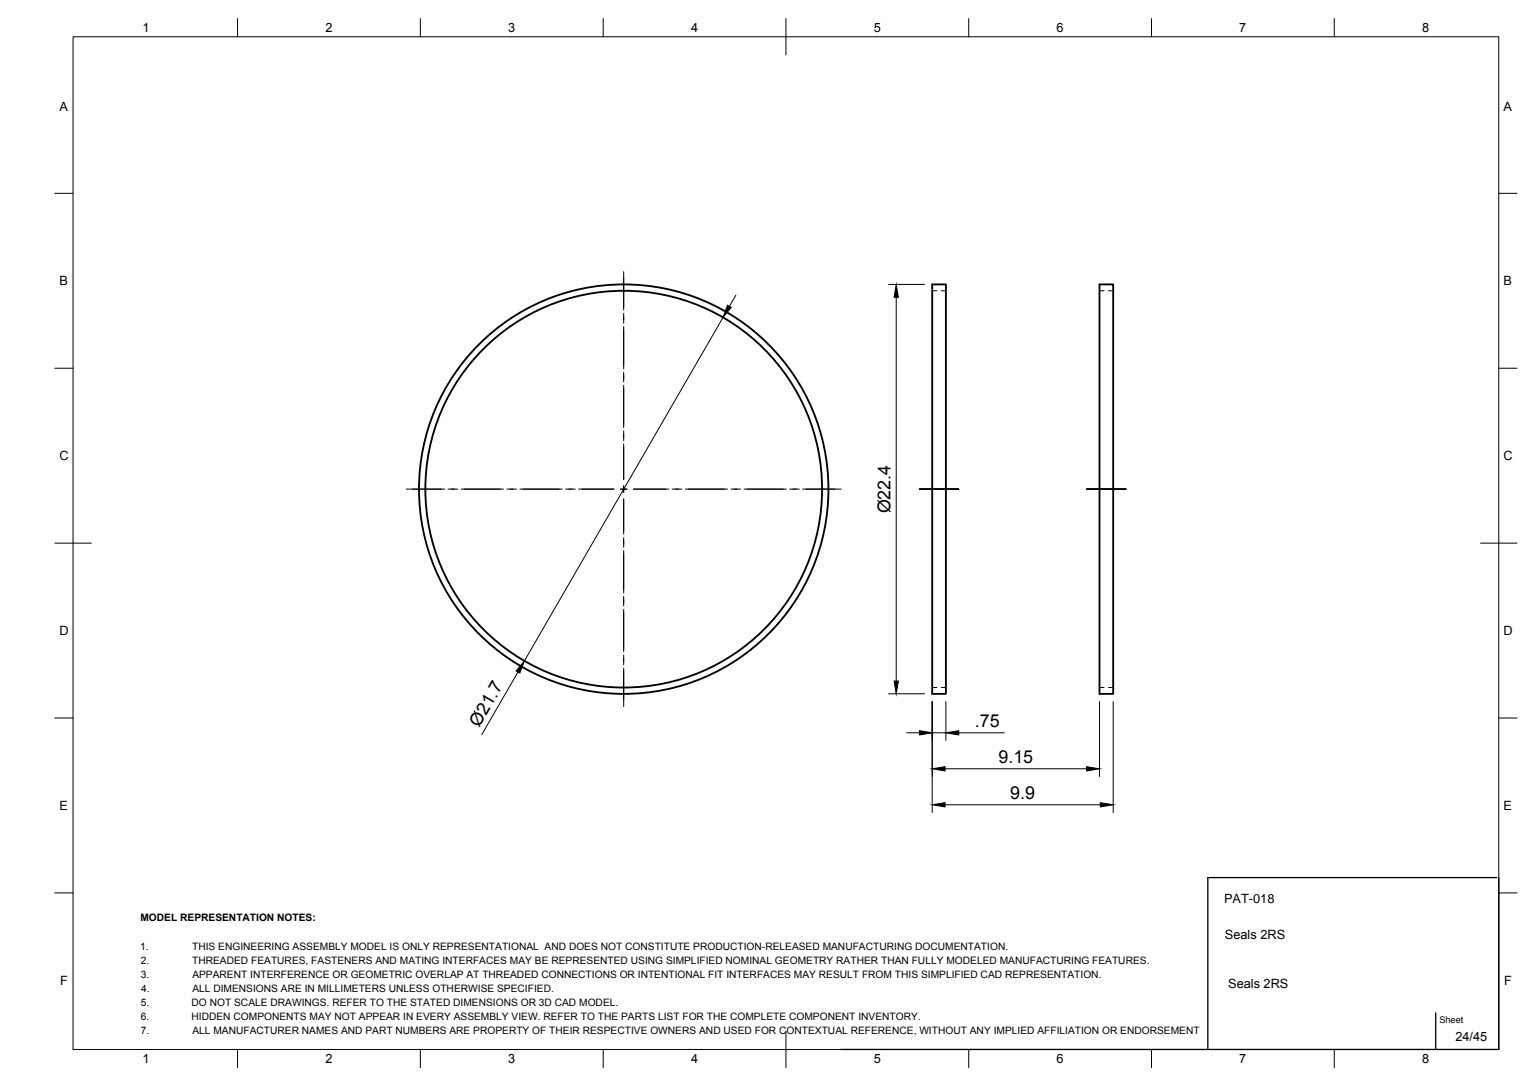
ISO-10303-21;
HEADER;
/* Generated by software containing ST-Developer
 * from STEP Tools, Inc. (www.steptools.com) 
 */

FILE_DESCRIPTION(
/* description */ ('Cam-driven reciprocating slide'),
/* implementation_level */ '2;1');

FILE_NAME(
/* name */ 'Seals 2RS.step',
/* time_stamp */ '2026-10-28T03:25:20-07:00',
/* author */ (''),
/* organization */ (''),
/* preprocessor_version */ 'ST-DEVELOPER v20.2',
/* originating_system */ 'Autodesk Translation Framework v15.17.0.0',
/* authorisation */ '');

FILE_SCHEMA (('AUTOMOTIVE_DESIGN { 1 0 10303 214 3 1 1 }'));
ENDSEC;

DATA;
#10=MECHANICAL_DESIGN_GEOMETRIC_PRESENTATION_REPRESENTATION('',(#445,#446),#13277);
#365=SHAPE_REPRESENTATION_RELATIONSHIP('SRR','None',#13459,#402);
#402=ADVANCED_BREP_SHAPE_REPRESENTATION('',(#489,#490),#13254);
#445=STYLED_ITEM('',(#13720),#489);
#446=STYLED_ITEM('',(#13720),#490);
#489=MANIFOLD_SOLID_BREP('Body1',#6421);
#490=MANIFOLD_SOLID_BREP('Body2',#6422);
#623=FACE_BOUND('',#1588,.T.);
#624=FACE_BOUND('',#1591,.T.);
#625=FACE_BOUND('',#1594,.T.);
#626=FACE_BOUND('',#1597,.T.);
#776=PLANE('',#7261);
#777=PLANE('',#7266);
#778=PLANE('',#7269);
#779=PLANE('',#7274);
#1092=FACE_OUTER_BOUND('',#1587,.T.);
#1093=FACE_OUTER_BOUND('',#1589,.T.);
#1094=FACE_OUTER_BOUND('',#1590,.T.);
#1095=FACE_OUTER_BOUND('',#1592,.T.);
#1096=FACE_OUTER_BOUND('',#1593,.T.);
#1097=FACE_OUTER_BOUND('',#1595,.T.);
#1098=FACE_OUTER_BOUND('',#1596,.T.);
#1099=FACE_OUTER_BOUND('',#1598,.T.);
#1587=EDGE_LOOP('',(#5182));
#1588=EDGE_LOOP('',(#5183));
#1589=EDGE_LOOP('',(#5184,#5185,#5186,#5187));
#1590=EDGE_LOOP('',(#5188));
#1591=EDGE_LOOP('',(#5189));
#1592=EDGE_LOOP('',(#5190,#5191,#5192,#5193));
#1593=EDGE_LOOP('',(#5194));
#1594=EDGE_LOOP('',(#5195));
#1595=EDGE_LOOP('',(#5196,#5197,#5198,#5199));
#1596=EDGE_LOOP('',(#5200));
#1597=EDGE_LOOP('',(#5201));
#1598=EDGE_LOOP('',(#5202,#5203,#5204,#5205));
#2044=LINE('',#12329,#2483);
#2045=LINE('',#12334,#2484);
#2046=LINE('',#12343,#2485);
#2047=LINE('',#12348,#2486);
#2483=VECTOR('',#8706,1.119765);
#2484=VECTOR('',#8713,1.085235);
#2485=VECTOR('',#8724,1.119765);
#2486=VECTOR('',#8731,1.085235);
#2908=CIRCLE('',#7262,1.119765);
#2909=CIRCLE('',#7263,1.085235);
#2910=CIRCLE('',#7265,1.119765);
#2911=CIRCLE('',#7267,1.085235);
#2912=CIRCLE('',#7270,1.119765);
#2913=CIRCLE('',#7271,1.085235);
#2914=CIRCLE('',#7273,1.119765);
#2915=CIRCLE('',#7275,1.085235);
#3325=VERTEX_POINT('',#12322);
#3326=VERTEX_POINT('',#12324);
#3327=VERTEX_POINT('',#12327);
#3328=VERTEX_POINT('',#12331);
#3329=VERTEX_POINT('',#12336);
#3330=VERTEX_POINT('',#12338);
#3331=VERTEX_POINT('',#12341);
#3332=VERTEX_POINT('',#12345);
#3981=EDGE_CURVE('',#3325,#3325,#2908,.T.);
#3982=EDGE_CURVE('',#3326,#3326,#2909,.T.);
#3983=EDGE_CURVE('',#3327,#3327,#2910,.T.);
#3984=EDGE_CURVE('',#3327,#3325,#2044,.T.);
#3985=EDGE_CURVE('',#3328,#3328,#2911,.T.);
#3986=EDGE_CURVE('',#3328,#3326,#2045,.T.);
#3987=EDGE_CURVE('',#3329,#3329,#2912,.T.);
#3988=EDGE_CURVE('',#3330,#3330,#2913,.T.);
#3989=EDGE_CURVE('',#3331,#3331,#2914,.T.);
#3990=EDGE_CURVE('',#3331,#3329,#2046,.T.);
#3991=EDGE_CURVE('',#3332,#3332,#2915,.T.);
#3992=EDGE_CURVE('',#3332,#3330,#2047,.T.);
#5182=ORIENTED_EDGE('',*,*,#3981,.F.);
#5183=ORIENTED_EDGE('',*,*,#3982,.T.);
#5184=ORIENTED_EDGE('',*,*,#3983,.F.);
#5185=ORIENTED_EDGE('',*,*,#3984,.T.);
#5186=ORIENTED_EDGE('',*,*,#3981,.T.);
#5187=ORIENTED_EDGE('',*,*,#3984,.F.);
#5188=ORIENTED_EDGE('',*,*,#3983,.T.);
#5189=ORIENTED_EDGE('',*,*,#3985,.F.);
#5190=ORIENTED_EDGE('',*,*,#3985,.T.);
#5191=ORIENTED_EDGE('',*,*,#3986,.T.);
#5192=ORIENTED_EDGE('',*,*,#3982,.F.);
#5193=ORIENTED_EDGE('',*,*,#3986,.F.);
#5194=ORIENTED_EDGE('',*,*,#3987,.F.);
#5195=ORIENTED_EDGE('',*,*,#3988,.T.);
#5196=ORIENTED_EDGE('',*,*,#3989,.F.);
#5197=ORIENTED_EDGE('',*,*,#3990,.T.);
#5198=ORIENTED_EDGE('',*,*,#3987,.T.);
#5199=ORIENTED_EDGE('',*,*,#3990,.F.);
#5200=ORIENTED_EDGE('',*,*,#3989,.T.);
#5201=ORIENTED_EDGE('',*,*,#3991,.F.);
#5202=ORIENTED_EDGE('',*,*,#3991,.T.);
#5203=ORIENTED_EDGE('',*,*,#3992,.T.);
#5204=ORIENTED_EDGE('',*,*,#3988,.F.);
#5205=ORIENTED_EDGE('',*,*,#3992,.F.);
#5967=CYLINDRICAL_SURFACE('',#7264,1.119765);
#5968=CYLINDRICAL_SURFACE('',#7268,1.085235);
#5969=CYLINDRICAL_SURFACE('',#7272,1.119765);
#5970=CYLINDRICAL_SURFACE('',#7276,1.085235);
#6210=ADVANCED_FACE('',(#1092,#623),#776,.T.);
#6211=ADVANCED_FACE('',(#1093),#5967,.T.);
#6212=ADVANCED_FACE('',(#1094,#624),#777,.T.);
#6213=ADVANCED_FACE('',(#1095),#5968,.F.);
#6214=ADVANCED_FACE('',(#1096,#625),#778,.T.);
#6215=ADVANCED_FACE('',(#1097),#5969,.T.);
#6216=ADVANCED_FACE('',(#1098,#626),#779,.T.);
#6217=ADVANCED_FACE('',(#1099),#5970,.F.);
#6421=CLOSED_SHELL('',(#6210,#6211,#6212,#6213));
#6422=CLOSED_SHELL('',(#6214,#6215,#6216,#6217));
#7260=AXIS2_PLACEMENT_3D('',#12320,#8694,#8695);
#7261=AXIS2_PLACEMENT_3D('',#12321,#8696,#8697);
#7262=AXIS2_PLACEMENT_3D('',#12323,#8698,#8699);
#7263=AXIS2_PLACEMENT_3D('',#12325,#8700,#8701);
#7264=AXIS2_PLACEMENT_3D('',#12326,#8702,#8703);
#7265=AXIS2_PLACEMENT_3D('',#12328,#8704,#8705);
#7266=AXIS2_PLACEMENT_3D('',#12330,#8707,#8708);
#7267=AXIS2_PLACEMENT_3D('',#12332,#8709,#8710);
#7268=AXIS2_PLACEMENT_3D('',#12333,#8711,#8712);
#7269=AXIS2_PLACEMENT_3D('',#12335,#8714,#8715);
#7270=AXIS2_PLACEMENT_3D('',#12337,#8716,#8717);
#7271=AXIS2_PLACEMENT_3D('',#12339,#8718,#8719);
#7272=AXIS2_PLACEMENT_3D('',#12340,#8720,#8721);
#7273=AXIS2_PLACEMENT_3D('',#12342,#8722,#8723);
#7274=AXIS2_PLACEMENT_3D('',#12344,#8725,#8726);
#7275=AXIS2_PLACEMENT_3D('',#12346,#8727,#8728);
#7276=AXIS2_PLACEMENT_3D('',#12347,#8729,#8730);
#8694=DIRECTION('axis',(0.,0.,1.));
#8695=DIRECTION('refdir',(1.,0.,0.));
#8696=DIRECTION('center_axis',(0.,1.,0.));
#8697=DIRECTION('ref_axis',(0.,0.,1.));
#8698=DIRECTION('center_axis',(0.,-1.,0.));
#8699=DIRECTION('ref_axis',(1.,0.,0.));
#8700=DIRECTION('center_axis',(0.,-1.,0.));
#8701=DIRECTION('ref_axis',(1.,0.,0.));
#8702=DIRECTION('center_axis',(0.,-1.,0.));
#8703=DIRECTION('ref_axis',(1.,0.,0.));
#8704=DIRECTION('center_axis',(0.,-1.,0.));
#8705=DIRECTION('ref_axis',(1.,0.,0.));
#8706=DIRECTION('',(0.,1.,0.));
#8707=DIRECTION('center_axis',(0.,-1.,0.));
#8708=DIRECTION('ref_axis',(0.,0.,-1.));
#8709=DIRECTION('center_axis',(0.,-1.,0.));
#8710=DIRECTION('ref_axis',(1.,0.,0.));
#8711=DIRECTION('center_axis',(0.,-1.,0.));
#8712=DIRECTION('ref_axis',(1.,0.,0.));
#8713=DIRECTION('',(0.,1.,0.));
#8714=DIRECTION('center_axis',(0.,1.,0.));
#8715=DIRECTION('ref_axis',(0.,0.,1.));
#8716=DIRECTION('center_axis',(0.,-1.,0.));
#8717=DIRECTION('ref_axis',(1.,0.,0.));
#8718=DIRECTION('center_axis',(0.,-1.,0.));
#8719=DIRECTION('ref_axis',(1.,0.,0.));
#8720=DIRECTION('center_axis',(0.,-1.,0.));
#8721=DIRECTION('ref_axis',(1.,0.,0.));
#8722=DIRECTION('center_axis',(0.,-1.,0.));
#8723=DIRECTION('ref_axis',(1.,0.,0.));
#8724=DIRECTION('',(0.,1.,0.));
#8725=DIRECTION('center_axis',(0.,-1.,0.));
#8726=DIRECTION('ref_axis',(0.,0.,-1.));
#8727=DIRECTION('center_axis',(0.,-1.,0.));
#8728=DIRECTION('ref_axis',(1.,0.,0.));
#8729=DIRECTION('center_axis',(0.,-1.,0.));
#8730=DIRECTION('ref_axis',(1.,0.,0.));
#8731=DIRECTION('',(0.,1.,0.));
#12320=CARTESIAN_POINT('',(0.,0.,0.));
#12321=CARTESIAN_POINT('Origin',(1.119765,0.495,0.));
#12322=CARTESIAN_POINT('',(-1.119765,0.495,-1.37131662304724E-16));
#12323=CARTESIAN_POINT('Origin',(0.,0.495,0.));
#12324=CARTESIAN_POINT('',(-1.085235,0.495,-1.32902956907268E-16));
#12325=CARTESIAN_POINT('Origin',(0.,0.495,0.));
#12326=CARTESIAN_POINT('Origin',(0.,0.4575,0.));
#12327=CARTESIAN_POINT('',(-1.119765,0.42,-1.37131662304724E-16));
#12328=CARTESIAN_POINT('Origin',(0.,0.42,0.));
#12329=CARTESIAN_POINT('',(-1.119765,0.4575,-1.37131662304724E-16));
#12330=CARTESIAN_POINT('Origin',(1.085235,0.42,0.));
#12331=CARTESIAN_POINT('',(-1.085235,0.42,-1.32902956907268E-16));
#12332=CARTESIAN_POINT('Origin',(0.,0.42,0.));
#12333=CARTESIAN_POINT('Origin',(0.,0.4575,0.));
#12334=CARTESIAN_POINT('',(-1.085235,0.4575,-1.32902956907268E-16));
#12335=CARTESIAN_POINT('Origin',(1.119765,-0.42,0.));
#12336=CARTESIAN_POINT('',(-1.119765,-0.42,-1.37131662304724E-16));
#12337=CARTESIAN_POINT('Origin',(0.,-0.42,0.));
#12338=CARTESIAN_POINT('',(-1.085235,-0.42,-1.32902956907268E-16));
#12339=CARTESIAN_POINT('Origin',(0.,-0.42,0.));
#12340=CARTESIAN_POINT('Origin',(0.,-0.4575,0.));
#12341=CARTESIAN_POINT('',(-1.119765,-0.495,-1.37131662304724E-16));
#12342=CARTESIAN_POINT('Origin',(0.,-0.495,0.));
#12343=CARTESIAN_POINT('',(-1.119765,-0.4575,-1.37131662304724E-16));
#12344=CARTESIAN_POINT('Origin',(1.085235,-0.495,0.));
#12345=CARTESIAN_POINT('',(-1.085235,-0.495,-1.32902956907268E-16));
#12346=CARTESIAN_POINT('Origin',(0.,-0.495,0.));
#12347=CARTESIAN_POINT('Origin',(0.,-0.4575,0.));
#12348=CARTESIAN_POINT('',(-1.085235,-0.4575,-1.32902956907268E-16));
#13210=UNCERTAINTY_MEASURE_WITH_UNIT(LENGTH_MEASURE(0.001),#13278,
'DISTANCE_ACCURACY_VALUE',
'Maximum model space distance between geometric entities at asserted c
onnectivities');
#13233=UNCERTAINTY_MEASURE_WITH_UNIT(LENGTH_MEASURE(0.001),#13278,
'DISTANCE_ACCURACY_VALUE',
'Maximum model space distance between geometric entities at asserted c
onnectivities');
#13254=(
GEOMETRIC_REPRESENTATION_CONTEXT(3)
GLOBAL_UNCERTAINTY_ASSIGNED_CONTEXT((#13210))
GLOBAL_UNIT_ASSIGNED_CONTEXT((#13278,#13280,#13281))
REPRESENTATION_CONTEXT('','3D')
);
#13277=(
GEOMETRIC_REPRESENTATION_CONTEXT(3)
GLOBAL_UNCERTAINTY_ASSIGNED_CONTEXT((#13233))
GLOBAL_UNIT_ASSIGNED_CONTEXT((#13278,#13280,#13281))
REPRESENTATION_CONTEXT('','3D')
);
#13278=(
LENGTH_UNIT()
NAMED_UNIT(*)
SI_UNIT(.CENTI.,.METRE.)
);
#13280=(
NAMED_UNIT(*)
PLANE_ANGLE_UNIT()
SI_UNIT($,.RADIAN.)
);
#13281=(
NAMED_UNIT(*)
SI_UNIT($,.STERADIAN.)
SOLID_ANGLE_UNIT()
);
#13302=SHAPE_DEFINITION_REPRESENTATION(#13345,#13459);
#13345=PRODUCT_DEFINITION_SHAPE('',$,#13503);
#13459=SHAPE_REPRESENTATION('',(#7260),#13254);
#13482=PRODUCT_DEFINITION_CONTEXT('part definition',#13613,'design');
#13503=PRODUCT_DEFINITION('Seals 2RS','Seals 2RS',#13546,#13482);
#13546=PRODUCT_DEFINITION_FORMATION('',$,#13635);
#13613=APPLICATION_CONTEXT(
'Core Data for Automotive Mechanical Design Process');
#13614=PRODUCT_CONTEXT('part definition',#13613,'mechanical');
#13635=PRODUCT('Seals 2RS','Seals 2RS','Seals 2RS',(#13614));
#13714=COLOUR_RGB('Grey',0.48,0.52,0.57);
#13715=FILL_AREA_STYLE_COLOUR('',#13714);
#13716=FILL_AREA_STYLE('',(#13715));
#13717=SURFACE_STYLE_FILL_AREA(#13716);
#13718=SURFACE_SIDE_STYLE('',(#13717));
#13719=SURFACE_STYLE_USAGE(.BOTH.,#13718);
#13720=PRESENTATION_STYLE_ASSIGNMENT((#13719));
ENDSEC;
END-ISO-10303-21;
